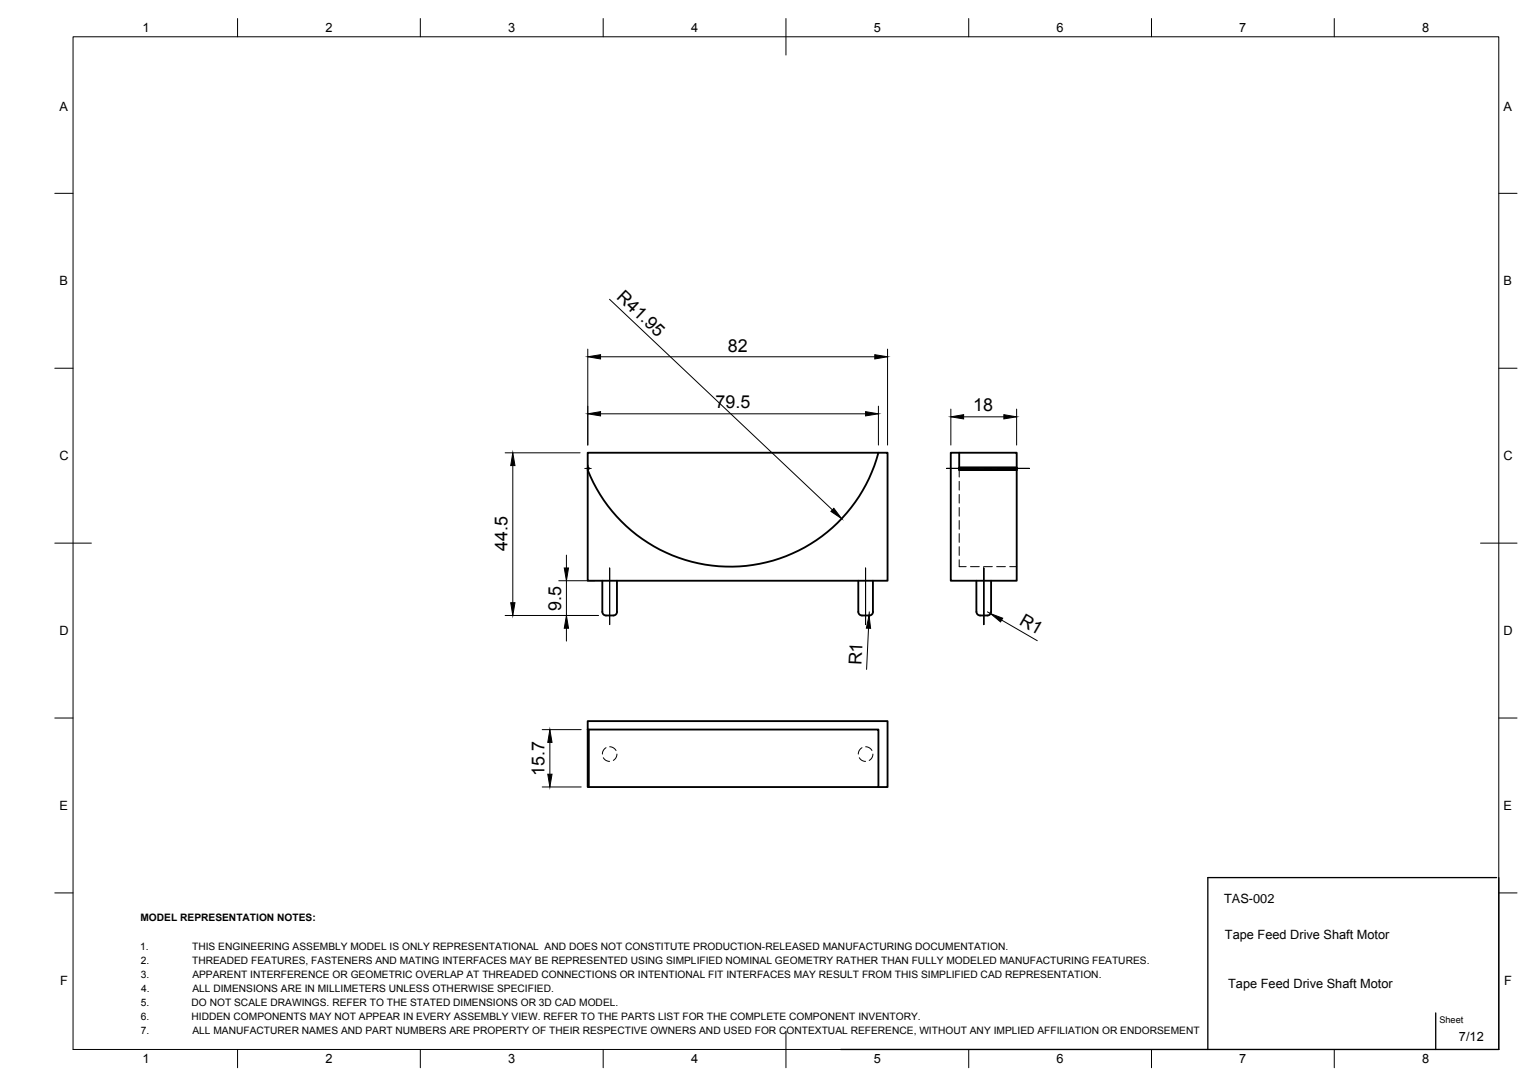
ISO-10303-21;
HEADER;
/* Generated by software containing ST-Developer
 * from STEP Tools, Inc. (www.steptools.com) 
 */

FILE_DESCRIPTION(
/* description */ ('STEP AP214'),
/* implementation_level */ '2;1');

FILE_NAME(
/* name */ 'Tape Feed Drive Shaft Motor.step',
/* time_stamp */ '2026-11-04T19:38:14-08:00',
/* author */ (''),
/* organization */ (''),
/* preprocessor_version */ 'ST-DEVELOPER v20.2',
/* originating_system */ 'Autodesk Translation Framework v15.17.0.0',
/* authorisation */ '');

FILE_SCHEMA (('AUTOMOTIVE_DESIGN { 1 0 10303 214 3 1 1 }'));
ENDSEC;

DATA;
#10=MECHANICAL_DESIGN_GEOMETRIC_PRESENTATION_REPRESENTATION('',(#474),#36668);
#409=(
BOUNDED_SURFACE()
B_SPLINE_SURFACE(2,2,((#27320,#27321,#27322,#27323,#27324,#27325,#27326,
#27327,#27328),(#27329,#27330,#27331,#27332,#27333,#27334,#27335,#27336,
#27337),(#27338,#27339,#27340,#27341,#27342,#27343,#27344,#27345,#27346)),
 .UNSPECIFIED.,.F.,.T.,.F.)
B_SPLINE_SURFACE_WITH_KNOTS((3,3),(3,2,2,2,3),(-7.86407345739089E-15,1.57079632679491),
(-3.14159265358979,-1.5707963267949,0.,1.5707963267949,3.14159265358979),
 .UNSPECIFIED.)
GEOMETRIC_REPRESENTATION_ITEM()
RATIONAL_B_SPLINE_SURFACE(((1.,0.707106781186548,1.,0.707106781186548,1.,
0.707106781186548,1.,0.707106781186548,1.),(0.707106781186533,0.499999999999989,
0.707106781186533,0.499999999999989,0.707106781186533,0.499999999999989,
0.707106781186533,0.499999999999989,0.707106781186533),(1.,0.707106781186548,
1.,0.707106781186548,1.,0.707106781186548,1.,0.707106781186548,1.)))
REPRESENTATION_ITEM('')
SURFACE()
);
#410=(
BOUNDED_SURFACE()
B_SPLINE_SURFACE(2,2,((#27354,#27355,#27356,#27357,#27358,#27359,#27360,
#27361,#27362),(#27363,#27364,#27365,#27366,#27367,#27368,#27369,#27370,
#27371),(#27372,#27373,#27374,#27375,#27376,#27377,#27378,#27379,#27380)),
 .UNSPECIFIED.,.F.,.T.,.F.)
B_SPLINE_SURFACE_WITH_KNOTS((3,3),(3,2,2,2,3),(-7.86407345739086E-15,1.57079632679491),
(-3.14159265358979,-1.5707963267949,0.,1.5707963267949,3.14159265358979),
 .UNSPECIFIED.)
GEOMETRIC_REPRESENTATION_ITEM()
RATIONAL_B_SPLINE_SURFACE(((1.,0.707106781186548,1.,0.707106781186548,1.,
0.707106781186548,1.,0.707106781186548,1.),(0.707106781186533,0.499999999999989,
0.707106781186533,0.499999999999989,0.707106781186533,0.499999999999989,
0.707106781186533,0.499999999999989,0.707106781186533),(1.,0.707106781186548,
1.,0.707106781186548,1.,0.707106781186548,1.,0.707106781186548,1.)))
REPRESENTATION_ITEM('')
SURFACE()
);
#454=SHAPE_REPRESENTATION_RELATIONSHIP('SRR','None',#36710,#464);
#464=ADVANCED_BREP_SHAPE_REPRESENTATION('',(#484),#36662);
#474=STYLED_ITEM('',(#36769),#484);
#484=MANIFOLD_SOLID_BREP('Body1',#17797);
#614=CYLINDRICAL_SURFACE('',#18727,0.233315989528693);
#615=CYLINDRICAL_SURFACE('',#18730,41.9475849136215);
#616=CYLINDRICAL_SURFACE('',#18743,2.);
#617=CYLINDRICAL_SURFACE('',#18746,2.);
#925=FACE_BOUND('',#3049,.T.);
#926=FACE_BOUND('',#3050,.T.);
#1339=CIRCLE('',#18728,0.233315989528693);
#1340=CIRCLE('',#18729,0.233315989528693);
#1341=CIRCLE('',#18731,41.9475849136215);
#1342=CIRCLE('',#18732,41.9475849136215);
#1343=CIRCLE('',#18734,1.);
#1344=CIRCLE('',#18735,1.);
#1345=CIRCLE('',#18736,2.);
#1346=CIRCLE('',#18737,2.);
#1347=CIRCLE('',#18738,1.);
#1348=CIRCLE('',#18739,1.);
#1349=CIRCLE('',#18740,2.);
#1350=CIRCLE('',#18741,2.);
#1351=CIRCLE('',#18744,2.);
#1352=CIRCLE('',#18747,2.);
#1957=FACE_OUTER_BOUND('',#3037,.T.);
#1958=FACE_OUTER_BOUND('',#3038,.T.);
#1959=FACE_OUTER_BOUND('',#3039,.T.);
#1960=FACE_OUTER_BOUND('',#3040,.T.);
#1961=FACE_OUTER_BOUND('',#3041,.T.);
#1962=FACE_OUTER_BOUND('',#3042,.T.);
#1963=FACE_OUTER_BOUND('',#3043,.T.);
#1964=FACE_OUTER_BOUND('',#3044,.T.);
#1965=FACE_OUTER_BOUND('',#3045,.T.);
#1966=FACE_OUTER_BOUND('',#3046,.T.);
#1967=FACE_OUTER_BOUND('',#3047,.T.);
#1968=FACE_OUTER_BOUND('',#3048,.T.);
#1969=FACE_OUTER_BOUND('',#3051,.T.);
#1970=FACE_OUTER_BOUND('',#3052,.T.);
#1971=FACE_OUTER_BOUND('',#3053,.T.);
#1972=FACE_OUTER_BOUND('',#3054,.T.);
#3037=EDGE_LOOP('',(#13642,#13643,#13644,#13645));
#3038=EDGE_LOOP('',(#13646,#13647,#13648,#13649));
#3039=EDGE_LOOP('',(#13650,#13651,#13652,#13653,#13654));
#3040=EDGE_LOOP('',(#13655,#13656,#13657,#13658,#13659));
#3041=EDGE_LOOP('',(#13660,#13661,#13662,#13663,#13664));
#3042=EDGE_LOOP('',(#13665));
#3043=EDGE_LOOP('',(#13666,#13667,#13668,#13669,#13670));
#3044=EDGE_LOOP('',(#13671));
#3045=EDGE_LOOP('',(#13672,#13673,#13674,#13675,#13676));
#3046=EDGE_LOOP('',(#13677,#13678));
#3047=EDGE_LOOP('',(#13679,#13680,#13681,#13682));
#3048=EDGE_LOOP('',(#13683,#13684,#13685,#13686));
#3049=EDGE_LOOP('',(#13687));
#3050=EDGE_LOOP('',(#13688));
#3051=EDGE_LOOP('',(#13689,#13690,#13691,#13692));
#3052=EDGE_LOOP('',(#13693,#13694,#13695,#13696,#13697,#13698));
#3053=EDGE_LOOP('',(#13699,#13700,#13701,#13702,#13703,#13704,#13705,#13706,
#13707,#13708));
#3054=EDGE_LOOP('',(#13709,#13710,#13711,#13712,#13713));
#4372=LINE('',#27302,#6082);
#4373=LINE('',#27305,#6083);
#4374=LINE('',#27311,#6084);
#4375=LINE('',#27314,#6085);
#4376=LINE('',#27317,#6086);
#4377=LINE('',#27318,#6087);
#4378=LINE('',#27319,#6088);
#4379=LINE('',#27392,#6089);
#4380=LINE('',#27397,#6090);
#4381=LINE('',#27399,#6091);
#4382=LINE('',#27403,#6092);
#4383=LINE('',#27405,#6093);
#4384=LINE('',#27407,#6094);
#4385=LINE('',#27408,#6095);
#4386=LINE('',#27412,#6096);
#4387=LINE('',#27413,#6097);
#4388=LINE('',#27414,#6098);
#4389=LINE('',#27417,#6099);
#4390=LINE('',#27418,#6100);
#4391=LINE('',#27420,#6101);
#4392=LINE('',#27421,#6102);
#4393=LINE('',#27423,#6103);
#6082=VECTOR('',#21852,1000.);
#6083=VECTOR('',#21855,1000.);
#6084=VECTOR('',#21860,1000.);
#6085=VECTOR('',#21863,1000.);
#6086=VECTOR('',#21866,1000.);
#6087=VECTOR('',#21867,1000.);
#6088=VECTOR('',#21868,1000.);
#6089=VECTOR('',#21891,2.);
#6090=VECTOR('',#21898,2.);
#6091=VECTOR('',#21901,1000.);
#6092=VECTOR('',#21904,1000.);
#6093=VECTOR('',#21905,1000.);
#6094=VECTOR('',#21906,1000.);
#6095=VECTOR('',#21907,1000.);
#6096=VECTOR('',#21910,1000.);
#6097=VECTOR('',#21911,1000.);
#6098=VECTOR('',#21912,1000.);
#6099=VECTOR('',#21915,1000.);
#6100=VECTOR('',#21916,1000.);
#6101=VECTOR('',#21919,1000.);
#6102=VECTOR('',#21920,1000.);
#6103=VECTOR('',#21923,1000.);
#7783=VERTEX_POINT('',#27298);
#7784=VERTEX_POINT('',#27299);
#7785=VERTEX_POINT('',#27301);
#7786=VERTEX_POINT('',#27303);
#7787=VERTEX_POINT('',#27307);
#7788=VERTEX_POINT('',#27308);
#7789=VERTEX_POINT('',#27310);
#7790=VERTEX_POINT('',#27312);
#7791=VERTEX_POINT('',#27316);
#7792=VERTEX_POINT('',#27347);
#7793=VERTEX_POINT('',#27349);
#7794=VERTEX_POINT('',#27351);
#7795=VERTEX_POINT('',#27381);
#7796=VERTEX_POINT('',#27383);
#7797=VERTEX_POINT('',#27385);
#7798=VERTEX_POINT('',#27390);
#7799=VERTEX_POINT('',#27395);
#7800=VERTEX_POINT('',#27401);
#7801=VERTEX_POINT('',#27402);
#7802=VERTEX_POINT('',#27404);
#7803=VERTEX_POINT('',#27406);
#7804=VERTEX_POINT('',#27410);
#7805=VERTEX_POINT('',#27411);
#7806=VERTEX_POINT('',#27416);
#9873=EDGE_CURVE('',#7783,#7784,#1339,.T.);
#9874=EDGE_CURVE('',#7783,#7785,#4372,.T.);
#9875=EDGE_CURVE('',#7785,#7786,#1340,.T.);
#9876=EDGE_CURVE('',#7784,#7786,#4373,.T.);
#9877=EDGE_CURVE('',#7787,#7788,#1341,.T.);
#9878=EDGE_CURVE('',#7789,#7788,#4374,.T.);
#9879=EDGE_CURVE('',#7790,#7789,#1342,.T.);
#9880=EDGE_CURVE('',#7787,#7790,#4375,.T.);
#9881=EDGE_CURVE('',#7789,#7791,#4376,.T.);
#9882=EDGE_CURVE('',#7791,#7783,#4377,.T.);
#9883=EDGE_CURVE('',#7790,#7784,#4378,.T.);
#9884=EDGE_CURVE('',#7792,#7792,#1343,.T.);
#9885=EDGE_CURVE('',#7792,#7793,#1344,.T.);
#9886=EDGE_CURVE('',#7794,#7793,#1345,.T.);
#9887=EDGE_CURVE('',#7793,#7794,#1346,.T.);
#9888=EDGE_CURVE('',#7795,#7795,#1347,.T.);
#9889=EDGE_CURVE('',#7795,#7796,#1348,.T.);
#9890=EDGE_CURVE('',#7797,#7796,#1349,.T.);
#9891=EDGE_CURVE('',#7796,#7797,#1350,.T.);
#9892=EDGE_CURVE('',#7798,#7798,#1351,.T.);
#9893=EDGE_CURVE('',#7798,#7794,#4379,.T.);
#9894=EDGE_CURVE('',#7799,#7799,#1352,.T.);
#9895=EDGE_CURVE('',#7799,#7797,#4380,.T.);
#9896=EDGE_CURVE('',#7786,#7785,#4381,.T.);
#9897=EDGE_CURVE('',#7800,#7801,#4382,.T.);
#9898=EDGE_CURVE('',#7801,#7802,#4383,.T.);
#9899=EDGE_CURVE('',#7802,#7803,#4384,.T.);
#9900=EDGE_CURVE('',#7803,#7800,#4385,.T.);
#9901=EDGE_CURVE('',#7804,#7805,#4386,.T.);
#9902=EDGE_CURVE('',#7803,#7805,#4387,.T.);
#9903=EDGE_CURVE('',#7802,#7804,#4388,.T.);
#9904=EDGE_CURVE('',#7806,#7804,#4389,.T.);
#9905=EDGE_CURVE('',#7801,#7806,#4390,.T.);
#9906=EDGE_CURVE('',#7788,#7806,#4391,.T.);
#9907=EDGE_CURVE('',#7800,#7791,#4392,.T.);
#9908=EDGE_CURVE('',#7805,#7787,#4393,.T.);
#13642=ORIENTED_EDGE('',*,*,#9873,.F.);
#13643=ORIENTED_EDGE('',*,*,#9874,.T.);
#13644=ORIENTED_EDGE('',*,*,#9875,.T.);
#13645=ORIENTED_EDGE('',*,*,#9876,.F.);
#13646=ORIENTED_EDGE('',*,*,#9877,.T.);
#13647=ORIENTED_EDGE('',*,*,#9878,.F.);
#13648=ORIENTED_EDGE('',*,*,#9879,.F.);
#13649=ORIENTED_EDGE('',*,*,#9880,.F.);
#13650=ORIENTED_EDGE('',*,*,#9879,.T.);
#13651=ORIENTED_EDGE('',*,*,#9881,.T.);
#13652=ORIENTED_EDGE('',*,*,#9882,.T.);
#13653=ORIENTED_EDGE('',*,*,#9873,.T.);
#13654=ORIENTED_EDGE('',*,*,#9883,.F.);
#13655=ORIENTED_EDGE('',*,*,#9884,.F.);
#13656=ORIENTED_EDGE('',*,*,#9885,.T.);
#13657=ORIENTED_EDGE('',*,*,#9886,.F.);
#13658=ORIENTED_EDGE('',*,*,#9887,.F.);
#13659=ORIENTED_EDGE('',*,*,#9885,.F.);
#13660=ORIENTED_EDGE('',*,*,#9888,.F.);
#13661=ORIENTED_EDGE('',*,*,#9889,.T.);
#13662=ORIENTED_EDGE('',*,*,#9890,.F.);
#13663=ORIENTED_EDGE('',*,*,#9891,.F.);
#13664=ORIENTED_EDGE('',*,*,#9889,.F.);
#13665=ORIENTED_EDGE('',*,*,#9884,.T.);
#13666=ORIENTED_EDGE('',*,*,#9892,.T.);
#13667=ORIENTED_EDGE('',*,*,#9893,.T.);
#13668=ORIENTED_EDGE('',*,*,#9886,.T.);
#13669=ORIENTED_EDGE('',*,*,#9887,.T.);
#13670=ORIENTED_EDGE('',*,*,#9893,.F.);
#13671=ORIENTED_EDGE('',*,*,#9888,.T.);
#13672=ORIENTED_EDGE('',*,*,#9894,.T.);
#13673=ORIENTED_EDGE('',*,*,#9895,.T.);
#13674=ORIENTED_EDGE('',*,*,#9890,.T.);
#13675=ORIENTED_EDGE('',*,*,#9891,.T.);
#13676=ORIENTED_EDGE('',*,*,#9895,.F.);
#13677=ORIENTED_EDGE('',*,*,#9875,.F.);
#13678=ORIENTED_EDGE('',*,*,#9896,.F.);
#13679=ORIENTED_EDGE('',*,*,#9897,.T.);
#13680=ORIENTED_EDGE('',*,*,#9898,.T.);
#13681=ORIENTED_EDGE('',*,*,#9899,.T.);
#13682=ORIENTED_EDGE('',*,*,#9900,.T.);
#13683=ORIENTED_EDGE('',*,*,#9901,.T.);
#13684=ORIENTED_EDGE('',*,*,#9902,.F.);
#13685=ORIENTED_EDGE('',*,*,#9899,.F.);
#13686=ORIENTED_EDGE('',*,*,#9903,.T.);
#13687=ORIENTED_EDGE('',*,*,#9894,.F.);
#13688=ORIENTED_EDGE('',*,*,#9892,.F.);
#13689=ORIENTED_EDGE('',*,*,#9904,.T.);
#13690=ORIENTED_EDGE('',*,*,#9903,.F.);
#13691=ORIENTED_EDGE('',*,*,#9898,.F.);
#13692=ORIENTED_EDGE('',*,*,#9905,.T.);
#13693=ORIENTED_EDGE('',*,*,#9881,.F.);
#13694=ORIENTED_EDGE('',*,*,#9878,.T.);
#13695=ORIENTED_EDGE('',*,*,#9906,.T.);
#13696=ORIENTED_EDGE('',*,*,#9905,.F.);
#13697=ORIENTED_EDGE('',*,*,#9897,.F.);
#13698=ORIENTED_EDGE('',*,*,#9907,.T.);
#13699=ORIENTED_EDGE('',*,*,#9908,.T.);
#13700=ORIENTED_EDGE('',*,*,#9880,.T.);
#13701=ORIENTED_EDGE('',*,*,#9883,.T.);
#13702=ORIENTED_EDGE('',*,*,#9876,.T.);
#13703=ORIENTED_EDGE('',*,*,#9896,.T.);
#13704=ORIENTED_EDGE('',*,*,#9874,.F.);
#13705=ORIENTED_EDGE('',*,*,#9882,.F.);
#13706=ORIENTED_EDGE('',*,*,#9907,.F.);
#13707=ORIENTED_EDGE('',*,*,#9900,.F.);
#13708=ORIENTED_EDGE('',*,*,#9902,.T.);
#13709=ORIENTED_EDGE('',*,*,#9877,.F.);
#13710=ORIENTED_EDGE('',*,*,#9908,.F.);
#13711=ORIENTED_EDGE('',*,*,#9901,.F.);
#13712=ORIENTED_EDGE('',*,*,#9904,.F.);
#13713=ORIENTED_EDGE('',*,*,#9906,.F.);
#16555=PLANE('',#18733);
#16556=PLANE('',#18742);
#16557=PLANE('',#18745);
#16558=PLANE('',#18748);
#16559=PLANE('',#18749);
#16560=PLANE('',#18750);
#16561=PLANE('',#18751);
#16562=PLANE('',#18752);
#16563=PLANE('',#18753);
#16564=PLANE('',#18754);
#17292=ADVANCED_FACE('',(#1957),#614,.T.);
#17293=ADVANCED_FACE('',(#1958),#615,.F.);
#17294=ADVANCED_FACE('',(#1959),#16555,.F.);
#17295=ADVANCED_FACE('',(#1960),#409,.F.);
#17296=ADVANCED_FACE('',(#1961),#410,.F.);
#17297=ADVANCED_FACE('',(#1962),#16556,.T.);
#17298=ADVANCED_FACE('',(#1963),#616,.T.);
#17299=ADVANCED_FACE('',(#1964),#16557,.T.);
#17300=ADVANCED_FACE('',(#1965),#617,.T.);
#17301=ADVANCED_FACE('',(#1966),#16558,.T.);
#17302=ADVANCED_FACE('',(#1967),#16559,.F.);
#17303=ADVANCED_FACE('',(#1968,#925,#926),#16560,.F.);
#17304=ADVANCED_FACE('',(#1969),#16561,.F.);
#17305=ADVANCED_FACE('',(#1970),#16562,.F.);
#17306=ADVANCED_FACE('',(#1971),#16563,.F.);
#17307=ADVANCED_FACE('',(#1972),#16564,.T.);
#17797=CLOSED_SHELL('',(#17292,#17293,#17294,#17295,#17296,#17297,#17298,
#17299,#17300,#17301,#17302,#17303,#17304,#17305,#17306,#17307));
#18726=AXIS2_PLACEMENT_3D('',#27296,#21846,#21847);
#18727=AXIS2_PLACEMENT_3D('',#27297,#21848,#21849);
#18728=AXIS2_PLACEMENT_3D('',#27300,#21850,#21851);
#18729=AXIS2_PLACEMENT_3D('',#27304,#21853,#21854);
#18730=AXIS2_PLACEMENT_3D('',#27306,#21856,#21857);
#18731=AXIS2_PLACEMENT_3D('',#27309,#21858,#21859);
#18732=AXIS2_PLACEMENT_3D('',#27313,#21861,#21862);
#18733=AXIS2_PLACEMENT_3D('',#27315,#21864,#21865);
#18734=AXIS2_PLACEMENT_3D('',#27348,#21869,#21870);
#18735=AXIS2_PLACEMENT_3D('',#27350,#21871,#21872);
#18736=AXIS2_PLACEMENT_3D('',#27352,#21873,#21874);
#18737=AXIS2_PLACEMENT_3D('',#27353,#21875,#21876);
#18738=AXIS2_PLACEMENT_3D('',#27382,#21877,#21878);
#18739=AXIS2_PLACEMENT_3D('',#27384,#21879,#21880);
#18740=AXIS2_PLACEMENT_3D('',#27386,#21881,#21882);
#18741=AXIS2_PLACEMENT_3D('',#27387,#21883,#21884);
#18742=AXIS2_PLACEMENT_3D('',#27388,#21885,#21886);
#18743=AXIS2_PLACEMENT_3D('',#27389,#21887,#21888);
#18744=AXIS2_PLACEMENT_3D('',#27391,#21889,#21890);
#18745=AXIS2_PLACEMENT_3D('',#27393,#21892,#21893);
#18746=AXIS2_PLACEMENT_3D('',#27394,#21894,#21895);
#18747=AXIS2_PLACEMENT_3D('',#27396,#21896,#21897);
#18748=AXIS2_PLACEMENT_3D('',#27398,#21899,#21900);
#18749=AXIS2_PLACEMENT_3D('',#27400,#21902,#21903);
#18750=AXIS2_PLACEMENT_3D('',#27409,#21908,#21909);
#18751=AXIS2_PLACEMENT_3D('',#27415,#21913,#21914);
#18752=AXIS2_PLACEMENT_3D('',#27419,#21917,#21918);
#18753=AXIS2_PLACEMENT_3D('',#27422,#21921,#21922);
#18754=AXIS2_PLACEMENT_3D('',#27424,#21924,#21925);
#21846=DIRECTION('axis',(0.,0.,1.));
#21847=DIRECTION('refdir',(1.,0.,0.));
#21848=DIRECTION('center_axis',(7.E-15,0.,1.));
#21849=DIRECTION('ref_axis',(-1.26181948956739E-14,-1.,8.76968602559222E-29));
#21850=DIRECTION('center_axis',(-7.E-15,0.,-1.));
#21851=DIRECTION('ref_axis',(-1.,0.,7.E-15));
#21852=DIRECTION('',(7.E-15,0.,1.));
#21853=DIRECTION('center_axis',(-7.E-15,0.,-1.));
#21854=DIRECTION('ref_axis',(-1.,0.,7.E-15));
#21855=DIRECTION('',(7.E-15,0.,1.));
#21856=DIRECTION('center_axis',(7.E-15,0.,1.));
#21857=DIRECTION('ref_axis',(-0.998223338976354,-0.0595832654601811,6.98756337283448E-15));
#21858=DIRECTION('center_axis',(7.E-15,0.,1.));
#21859=DIRECTION('ref_axis',(1.,0.,-7.E-15));
#21860=DIRECTION('',(7.E-15,0.,1.));
#21861=DIRECTION('center_axis',(7.E-15,0.,1.));
#21862=DIRECTION('ref_axis',(-1.,0.,7.E-15));
#21863=DIRECTION('',(-7.E-15,0.,-1.));
#21864=DIRECTION('center_axis',(-7.E-15,0.,-1.));
#21865=DIRECTION('ref_axis',(-1.,0.,7.E-15));
#21866=DIRECTION('',(0.,1.,0.));
#21867=DIRECTION('',(-1.,0.,7.E-15));
#21868=DIRECTION('',(1.,0.,-7.E-15));
#21869=DIRECTION('center_axis',(-1.,0.,7.E-15));
#21870=DIRECTION('ref_axis',(7.E-15,0.,1.));
#21871=DIRECTION('center_axis',(0.,-1.,0.));
#21872=DIRECTION('ref_axis',(-8.88178419700128E-15,0.,-1.));
#21873=DIRECTION('center_axis',(1.,0.,-7.E-15));
#21874=DIRECTION('ref_axis',(7.E-15,0.,1.));
#21875=DIRECTION('center_axis',(1.,0.,-7.E-15));
#21876=DIRECTION('ref_axis',(7.E-15,0.,1.));
#21877=DIRECTION('center_axis',(-1.,0.,7.E-15));
#21878=DIRECTION('ref_axis',(7.E-15,0.,1.));
#21879=DIRECTION('center_axis',(0.,-1.,0.));
#21880=DIRECTION('ref_axis',(-8.88178419700128E-15,0.,-1.));
#21881=DIRECTION('center_axis',(1.,0.,-7.E-15));
#21882=DIRECTION('ref_axis',(7.E-15,0.,1.));
#21883=DIRECTION('center_axis',(1.,0.,-7.E-15));
#21884=DIRECTION('ref_axis',(7.E-15,0.,1.));
#21885=DIRECTION('center_axis',(-1.,0.,7.E-15));
#21886=DIRECTION('ref_axis',(0.,1.,0.));
#21887=DIRECTION('center_axis',(1.,0.,-7.E-15));
#21888=DIRECTION('ref_axis',(-7.E-15,0.,-1.));
#21889=DIRECTION('center_axis',(-1.,0.,7.E-15));
#21890=DIRECTION('ref_axis',(-7.E-15,0.,-1.));
#21891=DIRECTION('',(-1.,0.,7.E-15));
#21892=DIRECTION('center_axis',(-1.,0.,7.E-15));
#21893=DIRECTION('ref_axis',(0.,1.,0.));
#21894=DIRECTION('center_axis',(1.,0.,-7.E-15));
#21895=DIRECTION('ref_axis',(-7.E-15,0.,-1.));
#21896=DIRECTION('center_axis',(-1.,0.,7.E-15));
#21897=DIRECTION('ref_axis',(-7.E-15,0.,-1.));
#21898=DIRECTION('',(-1.,0.,7.E-15));
#21899=DIRECTION('center_axis',(7.E-15,0.,1.));
#21900=DIRECTION('ref_axis',(0.,-1.,0.));
#21901=DIRECTION('',(1.,0.,-7.E-15));
#21902=DIRECTION('center_axis',(7.E-15,0.,1.));
#21903=DIRECTION('ref_axis',(0.,-1.,0.));
#21904=DIRECTION('',(0.,-1.,0.));
#21905=DIRECTION('',(-1.,0.,7.E-15));
#21906=DIRECTION('',(0.,1.,0.));
#21907=DIRECTION('',(1.,0.,-7.E-15));
#21908=DIRECTION('center_axis',(1.,0.,-7.E-15));
#21909=DIRECTION('ref_axis',(-7.E-15,0.,-1.));
#21910=DIRECTION('',(0.,1.,0.));
#21911=DIRECTION('',(7.E-15,0.,1.));
#21912=DIRECTION('',(7.E-15,0.,1.));
#21913=DIRECTION('center_axis',(0.,1.,0.));
#21914=DIRECTION('ref_axis',(-1.,0.,7.E-15));
#21915=DIRECTION('',(-1.,0.,7.E-15));
#21916=DIRECTION('',(7.E-15,0.,1.));
#21917=DIRECTION('center_axis',(-1.,0.,7.E-15));
#21918=DIRECTION('ref_axis',(0.,1.,0.));
#21919=DIRECTION('',(0.,-1.,0.));
#21920=DIRECTION('',(7.E-15,0.,1.));
#21921=DIRECTION('center_axis',(0.,-1.,0.));
#21922=DIRECTION('ref_axis',(7.E-15,0.,1.));
#21923=DIRECTION('',(1.,0.,-7.E-15));
#21924=DIRECTION('center_axis',(7.E-15,0.,1.));
#21925=DIRECTION('ref_axis',(0.,-1.,0.));
#27296=CARTESIAN_POINT('',(0.,0.,0.));
#27297=CARTESIAN_POINT('Origin',(-92.5471485639041,33.372246530613,196.800000000001));
#27298=CARTESIAN_POINT('',(-92.3230162611117,33.437062129158,196.800000000001));
#27299=CARTESIAN_POINT('',(-92.7712808666964,33.437062129158,196.800000000001));
#27300=CARTESIAN_POINT('Origin',(-92.5471485639041,33.372246530613,196.800000000001));
#27301=CARTESIAN_POINT('',(-92.3230162611116,33.437062129158,212.500000000001));
#27302=CARTESIAN_POINT('',(-92.3230162611117,33.437062129158,196.800000000001));
#27303=CARTESIAN_POINT('',(-92.7712808666963,33.437062129158,212.500000000001));
#27304=CARTESIAN_POINT('Origin',(-92.547148563904,33.372246530613,212.500000000001));
#27305=CARTESIAN_POINT('',(-92.7712808666964,33.437062129158,196.800000000001));
#27306=CARTESIAN_POINT('Origin',(-77.4703641348207,-5.5271886295165,196.800000000001));
#27307=CARTESIAN_POINT('',(-93.0069996425685,33.437062129158,212.500000000001));
#27308=CARTESIAN_POINT('',(-88.261699248228,-46.062937870842,212.500000000001));
#27309=CARTESIAN_POINT('Origin',(-77.4703641348205,-5.5271886295165,212.500000000001));
#27310=CARTESIAN_POINT('',(-88.2616992482281,-46.062937870842,196.800000000001));
#27311=CARTESIAN_POINT('',(-88.2616992482281,-46.062937870842,196.800000000001));
#27312=CARTESIAN_POINT('',(-93.0069996425686,33.437062129158,196.800000000001));
#27313=CARTESIAN_POINT('Origin',(-77.4703641348207,-5.5271886295165,196.800000000001));
#27314=CARTESIAN_POINT('',(-93.0069996425686,33.437062129158,196.800000000001));
#27315=CARTESIAN_POINT('Origin',(-77.4703641348207,-5.5271886295165,196.800000000001));
#27316=CARTESIAN_POINT('',(-88.2616992482281,33.437062129158,196.800000000001));
#27317=CARTESIAN_POINT('',(-88.2616992482281,33.437062129158,196.800000000001));
#27318=CARTESIAN_POINT('',(-88.2616992482281,33.437062129158,196.800000000001));
#27319=CARTESIAN_POINT('',(-88.2616992482281,33.437062129158,196.800000000001));
#27320=CARTESIAN_POINT('Ctrl Pts',(-131.761699248228,-42.562937870842,201.500000000001));
#27321=CARTESIAN_POINT('Ctrl Pts',(-131.761699248228,-44.562937870842,201.500000000001));
#27322=CARTESIAN_POINT('Ctrl Pts',(-131.761699248228,-44.562937870842,203.500000000001));
#27323=CARTESIAN_POINT('Ctrl Pts',(-131.761699248228,-44.562937870842,205.500000000001));
#27324=CARTESIAN_POINT('Ctrl Pts',(-131.761699248228,-42.562937870842,205.500000000001));
#27325=CARTESIAN_POINT('Ctrl Pts',(-131.761699248228,-40.562937870842,205.500000000001));
#27326=CARTESIAN_POINT('Ctrl Pts',(-131.761699248228,-40.562937870842,203.500000000001));
#27327=CARTESIAN_POINT('Ctrl Pts',(-131.761699248228,-40.562937870842,201.500000000001));
#27328=CARTESIAN_POINT('Ctrl Pts',(-131.761699248228,-42.562937870842,201.500000000001));
#27329=CARTESIAN_POINT('Ctrl Pts',(-132.761699248228,-42.562937870842,201.500000000001));
#27330=CARTESIAN_POINT('Ctrl Pts',(-132.761699248228,-44.562937870842,201.500000000001));
#27331=CARTESIAN_POINT('Ctrl Pts',(-132.761699248228,-44.562937870842,203.500000000001));
#27332=CARTESIAN_POINT('Ctrl Pts',(-132.761699248228,-44.562937870842,205.500000000001));
#27333=CARTESIAN_POINT('Ctrl Pts',(-132.761699248228,-42.562937870842,205.500000000001));
#27334=CARTESIAN_POINT('Ctrl Pts',(-132.761699248228,-40.562937870842,205.500000000001));
#27335=CARTESIAN_POINT('Ctrl Pts',(-132.761699248228,-40.562937870842,203.500000000001));
#27336=CARTESIAN_POINT('Ctrl Pts',(-132.761699248228,-40.562937870842,201.500000000001));
#27337=CARTESIAN_POINT('Ctrl Pts',(-132.761699248228,-42.562937870842,201.500000000001));
#27338=CARTESIAN_POINT('Ctrl Pts',(-132.761699248228,-42.562937870842,202.500000000001));
#27339=CARTESIAN_POINT('Ctrl Pts',(-132.761699248228,-43.562937870842,202.500000000001));
#27340=CARTESIAN_POINT('Ctrl Pts',(-132.761699248228,-43.562937870842,203.500000000001));
#27341=CARTESIAN_POINT('Ctrl Pts',(-132.761699248228,-43.562937870842,204.500000000001));
#27342=CARTESIAN_POINT('Ctrl Pts',(-132.761699248228,-42.562937870842,204.500000000001));
#27343=CARTESIAN_POINT('Ctrl Pts',(-132.761699248228,-41.562937870842,204.500000000001));
#27344=CARTESIAN_POINT('Ctrl Pts',(-132.761699248228,-41.562937870842,203.500000000001));
#27345=CARTESIAN_POINT('Ctrl Pts',(-132.761699248228,-41.562937870842,202.500000000001));
#27346=CARTESIAN_POINT('Ctrl Pts',(-132.761699248228,-42.562937870842,202.500000000001));
#27347=CARTESIAN_POINT('',(-132.761699248228,-42.562937870842,202.500000000001));
#27348=CARTESIAN_POINT('Origin',(-132.761699248228,-42.562937870842,203.500000000001));
#27349=CARTESIAN_POINT('',(-131.761699248228,-42.562937870842,201.500000000001));
#27350=CARTESIAN_POINT('Origin',(-131.761699248228,-42.562937870842,202.500000000001));
#27351=CARTESIAN_POINT('',(-131.761699248228,-42.562937870842,205.500000000001));
#27352=CARTESIAN_POINT('Origin',(-131.761699248228,-42.562937870842,203.500000000001));
#27353=CARTESIAN_POINT('Origin',(-131.761699248228,-42.562937870842,203.500000000001));
#27354=CARTESIAN_POINT('Ctrl Pts',(-131.761699248228,27.437062129158,201.500000000001));
#27355=CARTESIAN_POINT('Ctrl Pts',(-131.761699248228,25.437062129158,201.500000000001));
#27356=CARTESIAN_POINT('Ctrl Pts',(-131.761699248228,25.437062129158,203.500000000001));
#27357=CARTESIAN_POINT('Ctrl Pts',(-131.761699248228,25.437062129158,205.500000000001));
#27358=CARTESIAN_POINT('Ctrl Pts',(-131.761699248228,27.437062129158,205.500000000001));
#27359=CARTESIAN_POINT('Ctrl Pts',(-131.761699248228,29.437062129158,205.500000000001));
#27360=CARTESIAN_POINT('Ctrl Pts',(-131.761699248228,29.437062129158,203.500000000001));
#27361=CARTESIAN_POINT('Ctrl Pts',(-131.761699248228,29.437062129158,201.500000000001));
#27362=CARTESIAN_POINT('Ctrl Pts',(-131.761699248228,27.437062129158,201.500000000001));
#27363=CARTESIAN_POINT('Ctrl Pts',(-132.761699248228,27.437062129158,201.500000000001));
#27364=CARTESIAN_POINT('Ctrl Pts',(-132.761699248228,25.437062129158,201.500000000001));
#27365=CARTESIAN_POINT('Ctrl Pts',(-132.761699248228,25.437062129158,203.500000000001));
#27366=CARTESIAN_POINT('Ctrl Pts',(-132.761699248228,25.437062129158,205.500000000001));
#27367=CARTESIAN_POINT('Ctrl Pts',(-132.761699248228,27.437062129158,205.500000000001));
#27368=CARTESIAN_POINT('Ctrl Pts',(-132.761699248228,29.437062129158,205.500000000001));
#27369=CARTESIAN_POINT('Ctrl Pts',(-132.761699248228,29.437062129158,203.500000000001));
#27370=CARTESIAN_POINT('Ctrl Pts',(-132.761699248228,29.437062129158,201.500000000001));
#27371=CARTESIAN_POINT('Ctrl Pts',(-132.761699248228,27.437062129158,201.500000000001));
#27372=CARTESIAN_POINT('Ctrl Pts',(-132.761699248228,27.437062129158,202.500000000001));
#27373=CARTESIAN_POINT('Ctrl Pts',(-132.761699248228,26.437062129158,202.500000000001));
#27374=CARTESIAN_POINT('Ctrl Pts',(-132.761699248228,26.437062129158,203.500000000001));
#27375=CARTESIAN_POINT('Ctrl Pts',(-132.761699248228,26.437062129158,204.500000000001));
#27376=CARTESIAN_POINT('Ctrl Pts',(-132.761699248228,27.437062129158,204.500000000001));
#27377=CARTESIAN_POINT('Ctrl Pts',(-132.761699248228,28.437062129158,204.500000000001));
#27378=CARTESIAN_POINT('Ctrl Pts',(-132.761699248228,28.437062129158,203.500000000001));
#27379=CARTESIAN_POINT('Ctrl Pts',(-132.761699248228,28.437062129158,202.500000000001));
#27380=CARTESIAN_POINT('Ctrl Pts',(-132.761699248228,27.437062129158,202.500000000001));
#27381=CARTESIAN_POINT('',(-132.761699248228,27.437062129158,202.500000000001));
#27382=CARTESIAN_POINT('Origin',(-132.761699248228,27.437062129158,203.500000000001));
#27383=CARTESIAN_POINT('',(-131.761699248228,27.437062129158,201.500000000001));
#27384=CARTESIAN_POINT('Origin',(-131.761699248228,27.437062129158,202.500000000001));
#27385=CARTESIAN_POINT('',(-131.761699248228,27.437062129158,205.500000000001));
#27386=CARTESIAN_POINT('Origin',(-131.761699248228,27.437062129158,203.500000000001));
#27387=CARTESIAN_POINT('Origin',(-131.761699248228,27.437062129158,203.500000000001));
#27388=CARTESIAN_POINT('Origin',(-132.761699248228,-42.562937870842,203.500000000001));
#27389=CARTESIAN_POINT('Origin',(-132.761699248228,-42.562937870842,203.500000000001));
#27390=CARTESIAN_POINT('',(-123.261699248228,-42.562937870842,205.500000000001));
#27391=CARTESIAN_POINT('Origin',(-123.261699248228,-42.562937870842,203.500000000001));
#27392=CARTESIAN_POINT('',(-132.761699248228,-42.562937870842,205.500000000001));
#27393=CARTESIAN_POINT('Origin',(-132.761699248228,27.437062129158,203.500000000001));
#27394=CARTESIAN_POINT('Origin',(-132.761699248228,27.437062129158,203.500000000001));
#27395=CARTESIAN_POINT('',(-123.261699248228,27.437062129158,205.500000000001));
#27396=CARTESIAN_POINT('Origin',(-123.261699248228,27.437062129158,203.500000000001));
#27397=CARTESIAN_POINT('',(-132.761699248228,27.437062129158,205.500000000001));
#27398=CARTESIAN_POINT('Origin',(-88.261699248228,-48.562937870842,212.500000000001));
#27399=CARTESIAN_POINT('',(-88.261699248228,33.437062129158,212.500000000001));
#27400=CARTESIAN_POINT('Origin',(-88.2616992482281,-48.562937870842,194.500000000001));
#27401=CARTESIAN_POINT('',(-88.2616992482281,33.437062129158,194.500000000001));
#27402=CARTESIAN_POINT('',(-88.2616992482281,-48.562937870842,194.500000000001));
#27403=CARTESIAN_POINT('',(-88.2616992482281,-48.562937870842,194.500000000001));
#27404=CARTESIAN_POINT('',(-123.261699248228,-48.562937870842,194.500000000001));
#27405=CARTESIAN_POINT('',(-88.2616992482281,-48.562937870842,194.500000000001));
#27406=CARTESIAN_POINT('',(-123.261699248228,33.437062129158,194.500000000001));
#27407=CARTESIAN_POINT('',(-123.261699248228,-48.562937870842,194.500000000001));
#27408=CARTESIAN_POINT('',(-88.2616992482281,33.437062129158,194.500000000001));
#27409=CARTESIAN_POINT('Origin',(-123.261699248228,-48.562937870842,194.500000000001));
#27410=CARTESIAN_POINT('',(-123.261699248228,-48.562937870842,212.500000000001));
#27411=CARTESIAN_POINT('',(-123.261699248228,33.437062129158,212.500000000001));
#27412=CARTESIAN_POINT('',(-123.261699248228,-48.562937870842,212.500000000001));
#27413=CARTESIAN_POINT('',(-123.261699248228,33.437062129158,194.500000000001));
#27414=CARTESIAN_POINT('',(-123.261699248228,-48.562937870842,194.500000000001));
#27415=CARTESIAN_POINT('Origin',(-88.2616992482281,-48.562937870842,194.500000000001));
#27416=CARTESIAN_POINT('',(-88.261699248228,-48.562937870842,212.500000000001));
#27417=CARTESIAN_POINT('',(-88.261699248228,-48.562937870842,212.500000000001));
#27418=CARTESIAN_POINT('',(-88.2616992482281,-48.562937870842,194.500000000001));
#27419=CARTESIAN_POINT('Origin',(-88.2616992482281,-48.562937870842,194.500000000001));
#27420=CARTESIAN_POINT('',(-88.261699248228,-48.562937870842,212.500000000001));
#27421=CARTESIAN_POINT('',(-88.2616992482281,33.437062129158,194.500000000001));
#27422=CARTESIAN_POINT('Origin',(-88.2616992482281,33.437062129158,194.500000000001));
#27423=CARTESIAN_POINT('',(-88.261699248228,33.437062129158,212.500000000001));
#27424=CARTESIAN_POINT('Origin',(-88.261699248228,-48.562937870842,212.500000000001));
#36650=UNCERTAINTY_MEASURE_WITH_UNIT(LENGTH_MEASURE(0.01),#36669,
'DISTANCE_ACCURACY_VALUE',
'Maximum model space distance between geometric entities at asserted c
onnectivities');
#36656=UNCERTAINTY_MEASURE_WITH_UNIT(LENGTH_MEASURE(0.01),#36669,
'DISTANCE_ACCURACY_VALUE',
'Maximum model space distance between geometric entities at asserted c
onnectivities');
#36662=(
GEOMETRIC_REPRESENTATION_CONTEXT(3)
GLOBAL_UNCERTAINTY_ASSIGNED_CONTEXT((#36650))
GLOBAL_UNIT_ASSIGNED_CONTEXT((#36669,#36671,#36672))
REPRESENTATION_CONTEXT('','3D')
);
#36668=(
GEOMETRIC_REPRESENTATION_CONTEXT(3)
GLOBAL_UNCERTAINTY_ASSIGNED_CONTEXT((#36656))
GLOBAL_UNIT_ASSIGNED_CONTEXT((#36669,#36671,#36672))
REPRESENTATION_CONTEXT('','3D')
);
#36669=(
LENGTH_UNIT()
NAMED_UNIT(*)
SI_UNIT(.MILLI.,.METRE.)
);
#36671=(
NAMED_UNIT(*)
PLANE_ANGLE_UNIT()
SI_UNIT($,.RADIAN.)
);
#36672=(
NAMED_UNIT(*)
SI_UNIT($,.STERADIAN.)
SOLID_ANGLE_UNIT()
);
#36678=SHAPE_DEFINITION_REPRESENTATION(#36689,#36710);
#36689=PRODUCT_DEFINITION_SHAPE('',$,#36722);
#36710=SHAPE_REPRESENTATION('',(#18726),#36662);
#36716=PRODUCT_DEFINITION_CONTEXT('part definition',#36751,'design');
#36722=PRODUCT_DEFINITION('Tape Feed Drive Shaft Motor',
'Tape Feed Drive Shaft Motor',#36733,#36716);
#36733=PRODUCT_DEFINITION_FORMATION('',$,#36758);
#36751=APPLICATION_CONTEXT(
'Core Data for Automotive Mechanical Design Process');
#36752=PRODUCT_CONTEXT('part definition',#36751,'mechanical');
#36758=PRODUCT('Tape Feed Drive Shaft Motor',
'Tape Feed Drive Shaft Motor',$,(#36752));
#36769=PRESENTATION_STYLE_ASSIGNMENT((#36776));
#36776=SURFACE_STYLE_USAGE(.BOTH.,#36783);
#36783=SURFACE_SIDE_STYLE('',(#36790));
#36790=SURFACE_STYLE_FILL_AREA(#36797);
#36797=FILL_AREA_STYLE('Opaque(81,175,227)',(#36804));
#36804=FILL_AREA_STYLE_COLOUR('Opaque(81,175,227)',#36811);
#36811=COLOUR_RGB('Opaque(81,175,227)',0.317647058823529,0.686274509803922,
0.890196078431372);
ENDSEC;
END-ISO-10303-21;
